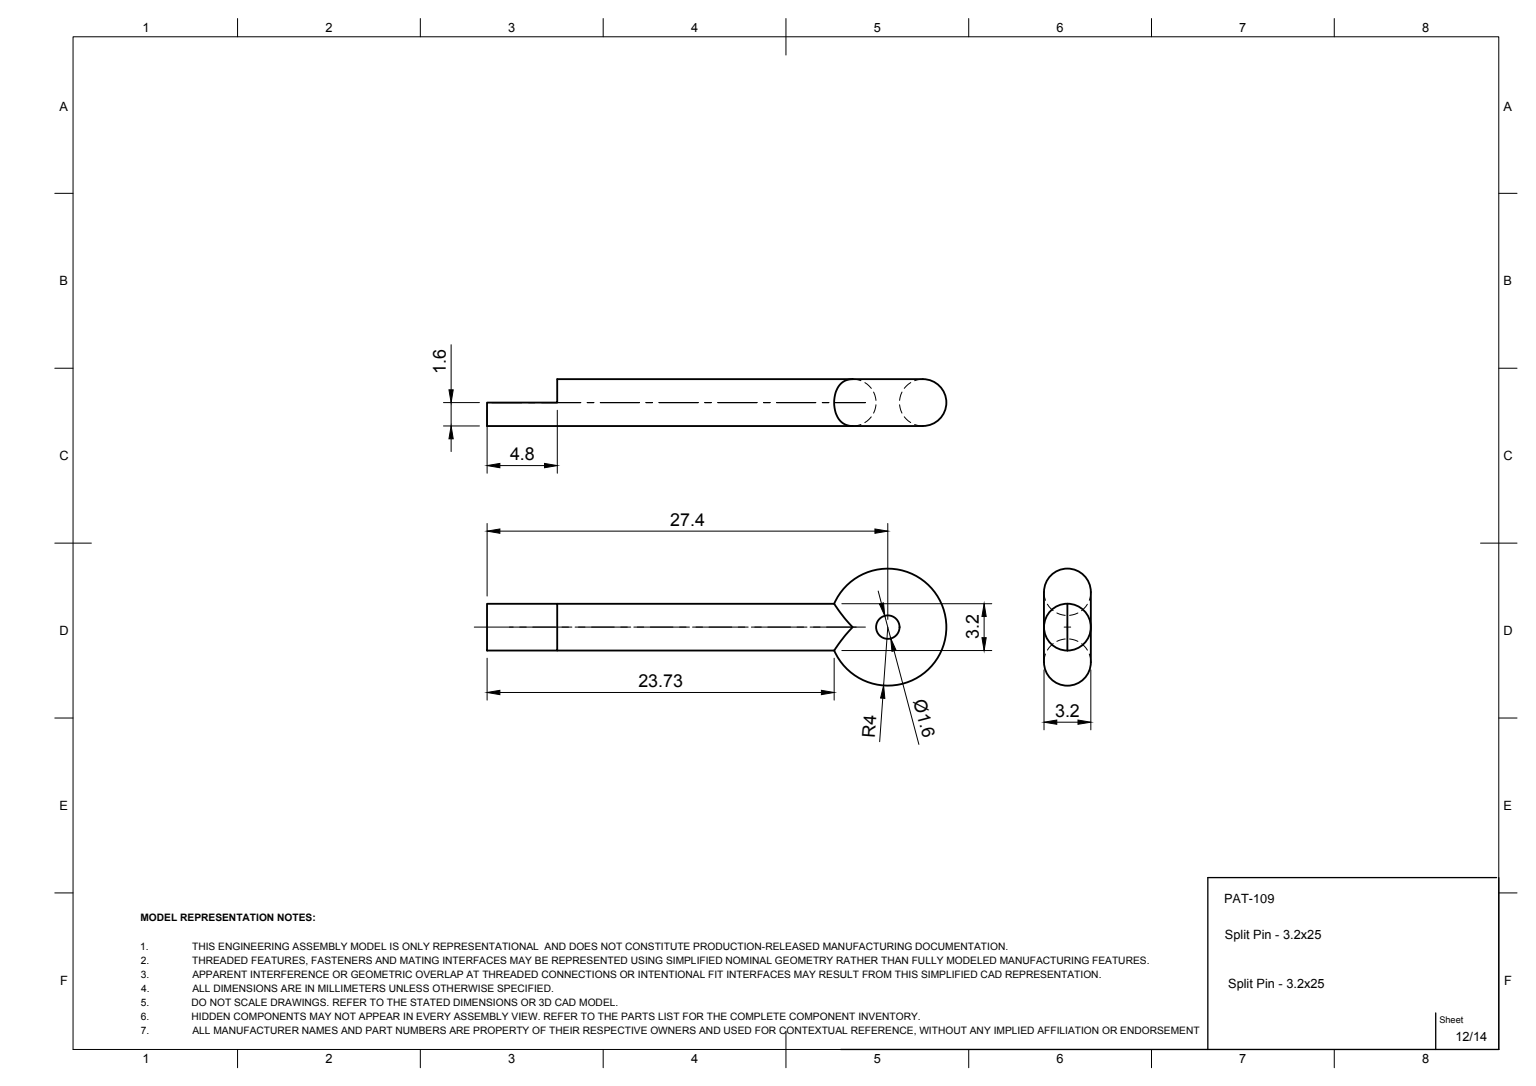
ISO-10303-21;
HEADER;
/* Generated by software containing ST-Developer
 * from STEP Tools, Inc. (www.steptools.com) 
 */

FILE_DESCRIPTION(
/* description */ ('Twin-shackle spreader bar'),
/* implementation_level */ '2;1');

FILE_NAME(
/* name */ 'Split Pin - 3.2x25.step',
/* time_stamp */ '2026-10-27T20:18:10-07:00',
/* author */ (''),
/* organization */ (''),
/* preprocessor_version */ 'ST-DEVELOPER v20.2',
/* originating_system */ 'Autodesk Translation Framework v15.17.0.0',
/* authorisation */ '');

FILE_SCHEMA (('AUTOMOTIVE_DESIGN { 1 0 10303 214 3 1 1 }'));
ENDSEC;

DATA;
#10=MECHANICAL_DESIGN_GEOMETRIC_PRESENTATION_REPRESENTATION('',(#163),#1829);
#11=TOROIDAL_SURFACE('',#1104,0.24,0.16);
#18=B_SPLINE_CURVE_WITH_KNOTS('',3,(#1720,#1721,#1722,#1723,#1724,#1725,
#1726,#1727,#1728,#1729,#1730,#1731,#1732,#1733,#1734,#1735,#1736,#1737,
#1738,#1739,#1740,#1741,#1742,#1743,#1744,#1745),.UNSPECIFIED.,.F.,.F.,
(4,2,2,2,2,2,2,2,2,2,2,2,4),(-0.000771405883143509,0.,0.0566386712389912,
0.124022719697233,0.181497823731714,0.241714216509916,0.290259365558526,
0.338804514607135,0.399020907385337,0.456496011419817,0.52388005987806,
0.580518731117043,0.581290137000192),.UNSPECIFIED.);
#19=B_SPLINE_CURVE_WITH_KNOTS('',3,(#1746,#1747,#1748,#1749,#1750,#1751,
#1752,#1753,#1754,#1755,#1756,#1757,#1758,#1759,#1760,#1761,#1762,#1763,
#1764,#1765,#1766,#1767,#1768,#1769,#1770,#1771),.UNSPECIFIED.,.F.,.F.,
(4,2,2,2,2,2,2,2,2,2,2,2,4),(-0.000771405883162359,0.,0.0566386712397236,
0.124022719698972,0.181497823734311,0.241714216513412,0.290259365562747,
0.338804514612082,0.399020907391184,0.456496011426523,0.523880059885771,
0.580518731125564,0.58129013700872),.UNSPECIFIED.);
#126=CIRCLE('',#1105,0.16);
#127=CIRCLE('',#1106,0.08);
#128=CIRCLE('',#1108,0.16);
#129=CIRCLE('',#1111,0.16);
#130=CIRCLE('',#1112,0.16);
#142=CYLINDRICAL_SURFACE('',#1110,0.16);
#149=SHAPE_REPRESENTATION_RELATIONSHIP('SRR','None',#1887,#156);
#156=ADVANCED_BREP_SHAPE_REPRESENTATION('',(#170),#1828);
#163=STYLED_ITEM('',(#1984),#170);
#170=MANIFOLD_SOLID_BREP('Body1',#943);
#185=FACE_BOUND('',#296,.T.);
#231=FACE_OUTER_BOUND('',#295,.T.);
#232=FACE_OUTER_BOUND('',#297,.T.);
#233=FACE_OUTER_BOUND('',#298,.T.);
#234=FACE_OUTER_BOUND('',#299,.T.);
#235=FACE_OUTER_BOUND('',#300,.T.);
#295=EDGE_LOOP('',(#828,#829,#830,#831));
#296=EDGE_LOOP('',(#832,#833));
#297=EDGE_LOOP('',(#834,#835));
#298=EDGE_LOOP('',(#836,#837,#838,#839));
#299=EDGE_LOOP('',(#840,#841,#842,#843,#844,#845,#846,#847,#848));
#300=EDGE_LOOP('',(#849,#850,#851));
#372=LINE('',#1776,#448);
#373=LINE('',#1779,#449);
#374=LINE('',#1781,#450);
#375=LINE('',#1782,#451);
#376=LINE('',#1786,#452);
#448=VECTOR('',#1376,1.);
#449=VECTOR('',#1379,1.);
#450=VECTOR('',#1380,1.);
#451=VECTOR('',#1381,1.);
#452=VECTOR('',#1386,0.16);
#517=VERTEX_POINT('',#1715);
#518=VERTEX_POINT('',#1718);
#519=VERTEX_POINT('',#1719);
#520=VERTEX_POINT('',#1773);
#521=VERTEX_POINT('',#1774);
#522=VERTEX_POINT('',#1778);
#523=VERTEX_POINT('',#1780);
#524=VERTEX_POINT('',#1784);
#622=EDGE_CURVE('',#517,#517,#126,.T.);
#623=EDGE_CURVE('',#517,#517,#127,.T.);
#624=EDGE_CURVE('',#518,#519,#18,.T.);
#625=EDGE_CURVE('',#519,#518,#19,.T.);
#626=EDGE_CURVE('',#520,#521,#128,.T.);
#627=EDGE_CURVE('',#520,#521,#372,.T.);
#628=EDGE_CURVE('',#521,#522,#373,.T.);
#629=EDGE_CURVE('',#523,#522,#374,.T.);
#630=EDGE_CURVE('',#520,#523,#375,.T.);
#631=EDGE_CURVE('',#524,#523,#129,.T.);
#632=EDGE_CURVE('',#524,#519,#376,.T.);
#633=EDGE_CURVE('',#522,#524,#130,.T.);
#828=ORIENTED_EDGE('',*,*,#622,.F.);
#829=ORIENTED_EDGE('',*,*,#623,.T.);
#830=ORIENTED_EDGE('',*,*,#622,.T.);
#831=ORIENTED_EDGE('',*,*,#623,.F.);
#832=ORIENTED_EDGE('',*,*,#624,.F.);
#833=ORIENTED_EDGE('',*,*,#625,.F.);
#834=ORIENTED_EDGE('',*,*,#626,.T.);
#835=ORIENTED_EDGE('',*,*,#627,.F.);
#836=ORIENTED_EDGE('',*,*,#627,.T.);
#837=ORIENTED_EDGE('',*,*,#628,.T.);
#838=ORIENTED_EDGE('',*,*,#629,.F.);
#839=ORIENTED_EDGE('',*,*,#630,.F.);
#840=ORIENTED_EDGE('',*,*,#626,.F.);
#841=ORIENTED_EDGE('',*,*,#630,.T.);
#842=ORIENTED_EDGE('',*,*,#631,.F.);
#843=ORIENTED_EDGE('',*,*,#632,.T.);
#844=ORIENTED_EDGE('',*,*,#625,.T.);
#845=ORIENTED_EDGE('',*,*,#624,.T.);
#846=ORIENTED_EDGE('',*,*,#632,.F.);
#847=ORIENTED_EDGE('',*,*,#633,.F.);
#848=ORIENTED_EDGE('',*,*,#628,.F.);
#849=ORIENTED_EDGE('',*,*,#633,.T.);
#850=ORIENTED_EDGE('',*,*,#631,.T.);
#851=ORIENTED_EDGE('',*,*,#629,.T.);
#884=PLANE('',#1107);
#885=PLANE('',#1109);
#886=PLANE('',#1113);
#932=ADVANCED_FACE('',(#231,#185),#11,.T.);
#933=ADVANCED_FACE('',(#232),#884,.F.);
#934=ADVANCED_FACE('',(#233),#885,.T.);
#935=ADVANCED_FACE('',(#234),#142,.T.);
#936=ADVANCED_FACE('',(#235),#886,.F.);
#943=CLOSED_SHELL('',(#932,#933,#934,#935,#936));
#1103=AXIS2_PLACEMENT_3D('',#1713,#1364,#1365);
#1104=AXIS2_PLACEMENT_3D('',#1714,#1366,#1367);
#1105=AXIS2_PLACEMENT_3D('',#1716,#1368,#1369);
#1106=AXIS2_PLACEMENT_3D('',#1717,#1370,#1371);
#1107=AXIS2_PLACEMENT_3D('',#1772,#1372,#1373);
#1108=AXIS2_PLACEMENT_3D('',#1775,#1374,#1375);
#1109=AXIS2_PLACEMENT_3D('',#1777,#1377,#1378);
#1110=AXIS2_PLACEMENT_3D('',#1783,#1382,#1383);
#1111=AXIS2_PLACEMENT_3D('',#1785,#1384,#1385);
#1112=AXIS2_PLACEMENT_3D('',#1787,#1387,#1388);
#1113=AXIS2_PLACEMENT_3D('',#1788,#1389,#1390);
#1364=DIRECTION('axis',(0.,0.,1.));
#1365=DIRECTION('refdir',(1.,0.,0.));
#1366=DIRECTION('center_axis',(-1.,0.,0.));
#1367=DIRECTION('ref_axis',(0.,0.,1.));
#1368=DIRECTION('center_axis',(0.,-1.,1.38777878078145E-16));
#1369=DIRECTION('ref_axis',(0.,-1.38777878078145E-16,-1.));
#1370=DIRECTION('center_axis',(1.,0.,0.));
#1371=DIRECTION('ref_axis',(0.,0.,1.));
#1372=DIRECTION('center_axis',(0.,1.,0.));
#1373=DIRECTION('ref_axis',(1.,0.,0.));
#1374=DIRECTION('center_axis',(0.,-1.,0.));
#1375=DIRECTION('ref_axis',(1.,0.,0.));
#1376=DIRECTION('',(0.,0.,1.));
#1377=DIRECTION('center_axis',(1.,0.,0.));
#1378=DIRECTION('ref_axis',(0.,0.,1.));
#1379=DIRECTION('',(0.,-1.,0.));
#1380=DIRECTION('',(0.,0.,1.));
#1381=DIRECTION('',(0.,-1.,0.));
#1382=DIRECTION('center_axis',(0.,-1.,0.));
#1383=DIRECTION('ref_axis',(1.,0.,0.));
#1384=DIRECTION('center_axis',(0.,-1.,0.));
#1385=DIRECTION('ref_axis',(1.,0.,0.));
#1386=DIRECTION('',(0.,1.,0.));
#1387=DIRECTION('center_axis',(0.,-1.,0.));
#1388=DIRECTION('ref_axis',(1.,0.,0.));
#1389=DIRECTION('center_axis',(0.,1.,0.));
#1390=DIRECTION('ref_axis',(1.,0.,0.));
#1713=CARTESIAN_POINT('',(0.,0.,0.));
#1714=CARTESIAN_POINT('Origin',(0.,0.24,0.));
#1715=CARTESIAN_POINT('',(-1.95943487863577E-17,0.24,-0.08));
#1716=CARTESIAN_POINT('Origin',(0.,0.24,-0.24));
#1717=CARTESIAN_POINT('Origin',(1.95943487863577E-17,0.24,0.));
#1718=CARTESIAN_POINT('',(0.16,-9.79717439317883E-18,1.46957615897682E-17));
#1719=CARTESIAN_POINT('',(-0.16,-9.79717439317883E-18,1.46957615897682E-17));
#1720=CARTESIAN_POINT('Ctrl Pts',(0.16,-9.79717439317883E-18,1.46957615897682E-17));
#1721=CARTESIAN_POINT('Ctrl Pts',(0.16,-0.000181822110339334,0.000181822110339339));
#1722=CARTESIAN_POINT('Ctrl Pts',(0.159999690069269,-0.000363540844324622,
0.000363747464878571));
#1723=CARTESIAN_POINT('Ctrl Pts',(0.159953479738417,-0.0138798266221246,
0.0139107352627986));
#1724=CARTESIAN_POINT('Ctrl Pts',(0.158232443771481,-0.0266233430820533,
0.0277973751356497));
#1725=CARTESIAN_POINT('Ctrl Pts',(0.149940017697612,-0.0530153061725048,
0.058442405232979));
#1726=CARTESIAN_POINT('Ctrl Pts',(0.142540414573103,-0.0662634124922917,
0.0751206840235135));
#1727=CARTESIAN_POINT('Ctrl Pts',(0.122571789881533,-0.0881367971480854,
0.104109120837503));
#1728=CARTESIAN_POINT('Ctrl Pts',(0.111018055346349,-0.0970398395589147,
0.116543563059122));
#1729=CARTESIAN_POINT('Ctrl Pts',(0.0824796164288417,-0.112218107746775,
0.138327679583944));
#1730=CARTESIAN_POINT('Ctrl Pts',(0.0655757961780097,-0.118179284966592,
0.147245809917584));
#1731=CARTESIAN_POINT('Ctrl Pts',(0.0318466054620204,-0.125035966654145,
0.157587272150341));
#1732=CARTESIAN_POINT('Ctrl Pts',(0.0160332282918615,-0.126606055596467,
0.16));
#1733=CARTESIAN_POINT('Ctrl Pts',(-0.0160332282918615,-0.126606055596467,
0.16));
#1734=CARTESIAN_POINT('Ctrl Pts',(-0.0318466054620203,-0.125035966654145,
0.157587272150341));
#1735=CARTESIAN_POINT('Ctrl Pts',(-0.0655757961780098,-0.118179284966592,
0.147245809917584));
#1736=CARTESIAN_POINT('Ctrl Pts',(-0.0824796164288418,-0.112218107746775,
0.138327679583943));
#1737=CARTESIAN_POINT('Ctrl Pts',(-0.111018055346349,-0.0970398395589147,
0.116543563059122));
#1738=CARTESIAN_POINT('Ctrl Pts',(-0.122571789881533,-0.0881367971480853,
0.104109120837503));
#1739=CARTESIAN_POINT('Ctrl Pts',(-0.142540414573103,-0.0662634124922916,
0.0751206840235135));
#1740=CARTESIAN_POINT('Ctrl Pts',(-0.149940017697612,-0.0530153061725049,
0.0584424052329791));
#1741=CARTESIAN_POINT('Ctrl Pts',(-0.158232443771481,-0.0266233430820551,
0.0277973751356518));
#1742=CARTESIAN_POINT('Ctrl Pts',(-0.159953479738417,-0.0138798266221373,
0.0139107352628116));
#1743=CARTESIAN_POINT('Ctrl Pts',(-0.159999690069269,-0.000363540844323022,
0.000363747464876927));
#1744=CARTESIAN_POINT('Ctrl Pts',(-0.16,-0.000181822110340974,0.000181822110340979));
#1745=CARTESIAN_POINT('Ctrl Pts',(-0.16,-9.79717439317883E-18,1.46957615897682E-17));
#1746=CARTESIAN_POINT('Ctrl Pts',(-0.16,-9.79717439317883E-18,1.46957615897682E-17));
#1747=CARTESIAN_POINT('Ctrl Pts',(-0.16,-0.000181822110343777,-0.000181822110343752));
#1748=CARTESIAN_POINT('Ctrl Pts',(-0.159999690069269,-0.000363540844320234,
-0.000363747464874079));
#1749=CARTESIAN_POINT('Ctrl Pts',(-0.159953479738416,-0.013879826622296,
-0.0139107352629724));
#1750=CARTESIAN_POINT('Ctrl Pts',(-0.158232443771474,-0.0266233430820775,
-0.0277973751356779));
#1751=CARTESIAN_POINT('Ctrl Pts',(-0.149940017697612,-0.053015306172505,
-0.0584424052329793));
#1752=CARTESIAN_POINT('Ctrl Pts',(-0.142540414573103,-0.0662634124922918,
-0.0751206840235137));
#1753=CARTESIAN_POINT('Ctrl Pts',(-0.122571789881533,-0.0881367971480854,
-0.104109120837503));
#1754=CARTESIAN_POINT('Ctrl Pts',(-0.111018055346349,-0.0970398395589147,
-0.116543563059122));
#1755=CARTESIAN_POINT('Ctrl Pts',(-0.0824796164288418,-0.112218107746775,
-0.138327679583943));
#1756=CARTESIAN_POINT('Ctrl Pts',(-0.0655757961780097,-0.118179284966592,
-0.147245809917584));
#1757=CARTESIAN_POINT('Ctrl Pts',(-0.0318466054620201,-0.125035966654145,
-0.157587272150341));
#1758=CARTESIAN_POINT('Ctrl Pts',(-0.0160332282918614,-0.126606055596467,
-0.16));
#1759=CARTESIAN_POINT('Ctrl Pts',(0.0160332282918614,-0.126606055596467,
-0.16));
#1760=CARTESIAN_POINT('Ctrl Pts',(0.0318466054620202,-0.125035966654145,
-0.157587272150341));
#1761=CARTESIAN_POINT('Ctrl Pts',(0.0655757961780098,-0.118179284966592,
-0.147245809917584));
#1762=CARTESIAN_POINT('Ctrl Pts',(0.0824796164288418,-0.112218107746775,
-0.138327679583943));
#1763=CARTESIAN_POINT('Ctrl Pts',(0.111018055346349,-0.0970398395589148,
-0.116543563059122));
#1764=CARTESIAN_POINT('Ctrl Pts',(0.122571789881533,-0.0881367971480855,
-0.104109120837504));
#1765=CARTESIAN_POINT('Ctrl Pts',(0.142540414573103,-0.0662634124922916,
-0.0751206840235135));
#1766=CARTESIAN_POINT('Ctrl Pts',(0.149940017697612,-0.0530153061725047,
-0.058442405232979));
#1767=CARTESIAN_POINT('Ctrl Pts',(0.158232443771478,-0.0266233430820626,
-0.0277973751356607));
#1768=CARTESIAN_POINT('Ctrl Pts',(0.159953479738417,-0.0138798266221904,
-0.0139107352628652));
#1769=CARTESIAN_POINT('Ctrl Pts',(0.159999690069269,-0.000363540844323479,
-0.000363747464877385));
#1770=CARTESIAN_POINT('Ctrl Pts',(0.16,-0.000181822110340484,-0.00018182211034046));
#1771=CARTESIAN_POINT('Ctrl Pts',(0.16,-9.79717439317883E-18,1.46957615897682E-17));
#1772=CARTESIAN_POINT('Origin',(0.08,-2.02,0.));
#1773=CARTESIAN_POINT('',(0.,-2.02,-0.16));
#1774=CARTESIAN_POINT('',(0.,-2.02,0.16));
#1775=CARTESIAN_POINT('Origin',(0.,-2.02,0.));
#1776=CARTESIAN_POINT('',(0.,-2.02,-0.08));
#1777=CARTESIAN_POINT('Origin',(0.,0.,-0.16));
#1778=CARTESIAN_POINT('',(0.,-2.5,0.16));
#1779=CARTESIAN_POINT('',(0.,0.,0.16));
#1780=CARTESIAN_POINT('',(0.,-2.5,-0.16));
#1781=CARTESIAN_POINT('',(0.,-2.5,-0.17));
#1782=CARTESIAN_POINT('',(0.,0.,-0.16));
#1783=CARTESIAN_POINT('Origin',(0.,0.,0.));
#1784=CARTESIAN_POINT('',(-0.16,-2.5,-1.95943487863577E-17));
#1785=CARTESIAN_POINT('Origin',(0.,-2.5,0.));
#1786=CARTESIAN_POINT('',(-0.16,0.,-1.95943487863577E-17));
#1787=CARTESIAN_POINT('Origin',(0.,-2.5,0.));
#1788=CARTESIAN_POINT('Origin',(-0.08,-2.5,0.));
#1816=UNCERTAINTY_MEASURE_WITH_UNIT(LENGTH_MEASURE(0.001),#1830,
'DISTANCE_ACCURACY_VALUE',
'Maximum model space distance between geometric entities at asserted c
onnectivities');
#1817=UNCERTAINTY_MEASURE_WITH_UNIT(LENGTH_MEASURE(0.001),#1830,
'DISTANCE_ACCURACY_VALUE',
'Maximum model space distance between geometric entities at asserted c
onnectivities');
#1828=(
GEOMETRIC_REPRESENTATION_CONTEXT(3)
GLOBAL_UNCERTAINTY_ASSIGNED_CONTEXT((#1816))
GLOBAL_UNIT_ASSIGNED_CONTEXT((#1830,#1832,#1833))
REPRESENTATION_CONTEXT('','3D')
);
#1829=(
GEOMETRIC_REPRESENTATION_CONTEXT(3)
GLOBAL_UNCERTAINTY_ASSIGNED_CONTEXT((#1817))
GLOBAL_UNIT_ASSIGNED_CONTEXT((#1830,#1832,#1833))
REPRESENTATION_CONTEXT('','3D')
);
#1830=(
LENGTH_UNIT()
NAMED_UNIT(*)
SI_UNIT(.CENTI.,.METRE.)
);
#1832=(
NAMED_UNIT(*)
PLANE_ANGLE_UNIT()
SI_UNIT($,.RADIAN.)
);
#1833=(
NAMED_UNIT(*)
SI_UNIT($,.STERADIAN.)
SOLID_ANGLE_UNIT()
);
#1844=SHAPE_DEFINITION_REPRESENTATION(#1859,#1887);
#1859=PRODUCT_DEFINITION_SHAPE('',$,#1899);
#1887=SHAPE_REPRESENTATION('',(#1103),#1828);
#1888=PRODUCT_DEFINITION_CONTEXT('part definition',#1923,'design');
#1899=PRODUCT_DEFINITION('Split Pin - 3.2x25','Split Pin - 3.2x25',#1910,
#1888);
#1910=PRODUCT_DEFINITION_FORMATION('',$,#1935);
#1923=APPLICATION_CONTEXT(
'Core Data for Automotive Mechanical Design Process');
#1924=PRODUCT_CONTEXT('part definition',#1923,'mechanical');
#1935=PRODUCT('Split Pin - 3.2x25','Split Pin - 3.2x25',
'Split Pin - 3.2x25',(#1924));
#1978=COLOUR_RGB('Grey',0.48,0.52,0.57);
#1979=FILL_AREA_STYLE_COLOUR('',#1978);
#1980=FILL_AREA_STYLE('',(#1979));
#1981=SURFACE_STYLE_FILL_AREA(#1980);
#1982=SURFACE_SIDE_STYLE('',(#1981));
#1983=SURFACE_STYLE_USAGE(.BOTH.,#1982);
#1984=PRESENTATION_STYLE_ASSIGNMENT((#1983));
ENDSEC;
END-ISO-10303-21;
